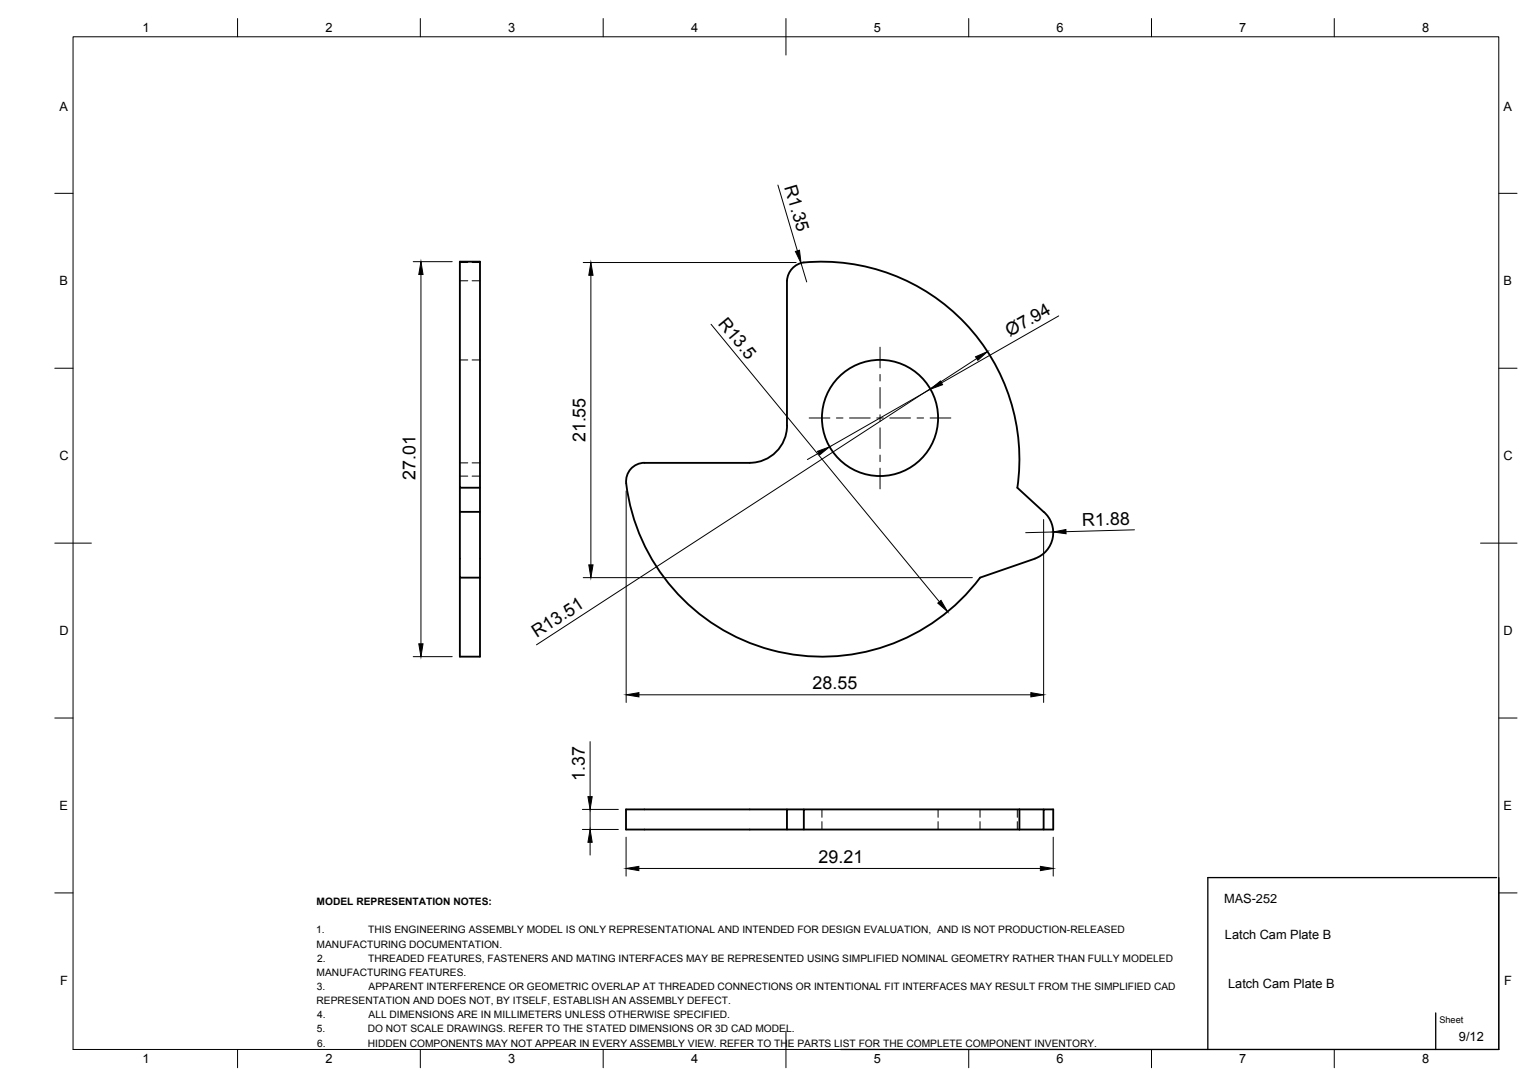
ISO-10303-21;
HEADER;
FILE_DESCRIPTION((''),'2;1');
FILE_NAME('Latch Cam Plate B.step','2026-10-06T07:01:46+05:00',(''),(''),'','','');
FILE_SCHEMA (('AUTOMOTIVE_DESIGN { 1 0 10303 214 3 1 1 }'));
ENDSEC;
DATA;
#10=MECHANICAL_DESIGN_GEOMETRIC_PRESENTATION_REPRESENTATION('',(#151),#11396);
#121=SHAPE_REPRESENTATION_RELATIONSHIP('SRR','None',#11468,#136) ;
#136=ADVANCED_BREP_SHAPE_REPRESENTATION('',(#166),#11394) ;
#151=STYLED_ITEM('',(#11552),#166) ;
#166=MANIFOLD_SOLID_BREP('Latch Cam Plate B',#5582) ;
#374=FACE_BOUND('',#1212,.T.) ;
#375=FACE_BOUND('',#1214,.T.) ;
#500=PLANE('',#6364) ;
#501=PLANE('',#6371) ;
#502=PLANE('',#6375) ;
#503=PLANE('',#6382) ;
#504=PLANE('',#6383) ;
#505=PLANE('',#6384) ;
#827=FACE_OUTER_BOUND('',#1200,.T.) ;
#828=FACE_OUTER_BOUND('',#1201,.T.) ;
#829=FACE_OUTER_BOUND('',#1202,.T.) ;
#830=FACE_OUTER_BOUND('',#1203,.T.) ;
#831=FACE_OUTER_BOUND('',#1204,.T.) ;
#832=FACE_OUTER_BOUND('',#1205,.T.) ;
#833=FACE_OUTER_BOUND('',#1206,.T.) ;
#834=FACE_OUTER_BOUND('',#1207,.T.) ;
#835=FACE_OUTER_BOUND('',#1208,.T.) ;
#836=FACE_OUTER_BOUND('',#1209,.T.) ;
#837=FACE_OUTER_BOUND('',#1210,.T.) ;
#838=FACE_OUTER_BOUND('',#1211,.T.) ;
#839=FACE_OUTER_BOUND('',#1213,.T.) ;
#1200=EDGE_LOOP('',(#5014,#5015,#5016,#5017)) ;
#1201=EDGE_LOOP('',(#5018,#5019,#5020,#5021)) ;
#1202=EDGE_LOOP('',(#5022,#5023,#5024,#5025)) ;
#1203=EDGE_LOOP('',(#5026,#5027,#5028,#5029)) ;
#1204=EDGE_LOOP('',(#5030,#5031,#5032,#5033)) ;
#1205=EDGE_LOOP('',(#5034,#5035,#5036,#5037)) ;
#1206=EDGE_LOOP('',(#5038,#5039,#5040,#5041)) ;
#1207=EDGE_LOOP('',(#5042,#5043,#5044,#5045)) ;
#1208=EDGE_LOOP('',(#5046,#5047,#5048,#5049)) ;
#1209=EDGE_LOOP('',(#5050,#5051,#5052,#5053)) ;
#1210=EDGE_LOOP('',(#5054,#5055,#5056,#5057)) ;
#1211=EDGE_LOOP('',(#5058,#5059,#5060,#5061,#5062,#5063,#5064,#5065,#5066,
#5067)) ;
#1212=EDGE_LOOP('',(#5068)) ;
#1213=EDGE_LOOP('',(#5069,#5070,#5071,#5072,#5073,#5074,#5075,#5076,#5077,
#5078)) ;
#1214=EDGE_LOOP('',(#5079)) ;
#1583=LINE('',#11263,#1966) ;
#1584=LINE('',#11270,#1967) ;
#1585=LINE('',#11273,#1968) ;
#1586=LINE('',#11276,#1969) ;
#1587=LINE('',#11278,#1970) ;
#1588=LINE('',#11279,#1971) ;
#1589=LINE('',#11285,#1972) ;
#1590=LINE('',#11291,#1973) ;
#1591=LINE('',#11294,#1974) ;
#1592=LINE('',#11296,#1975) ;
#1593=LINE('',#11297,#1976) ;
#1594=LINE('',#11303,#1977) ;
#1595=LINE('',#11306,#1978) ;
#1596=LINE('',#11308,#1979) ;
#1597=LINE('',#11309,#1980) ;
#1598=LINE('',#11315,#1981) ;
#1599=LINE('',#11321,#1982) ;
#1600=LINE('',#11323,#1983) ;
#1601=LINE('',#11324,#1984) ;
#1966=VECTOR('',#7997,3.97) ;
#1967=VECTOR('',#8004,10.) ;
#1968=VECTOR('',#8007,10.) ;
#1969=VECTOR('',#8010,10.) ;
#1970=VECTOR('',#8011,10.) ;
#1971=VECTOR('',#8012,10.) ;
#1972=VECTOR('',#8019,10.) ;
#1973=VECTOR('',#8026,10.) ;
#1974=VECTOR('',#8029,10.) ;
#1975=VECTOR('',#8030,10.) ;
#1976=VECTOR('',#8031,10.) ;
#1977=VECTOR('',#8038,10.) ;
#1978=VECTOR('',#8041,10.) ;
#1979=VECTOR('',#8042,10.) ;
#1980=VECTOR('',#8043,10.) ;
#1981=VECTOR('',#8050,10.) ;
#1982=VECTOR('',#8057,10.) ;
#1983=VECTOR('',#8060,10.) ;
#1984=VECTOR('',#8061,10.) ;
#2251=CIRCLE('',#6359,3.97) ;
#2252=CIRCLE('',#6360,3.97) ;
#2253=CIRCLE('',#6362,2.55000000000001) ;
#2254=CIRCLE('',#6363,2.55000000000001) ;
#2255=CIRCLE('',#6366,1.34638068543699) ;
#2256=CIRCLE('',#6367,1.34638068543699) ;
#2257=CIRCLE('',#6369,13.5130476224576) ;
#2258=CIRCLE('',#6370,13.5130476224576) ;
#2259=CIRCLE('',#6373,1.8820937834387) ;
#2260=CIRCLE('',#6374,1.8820937834387) ;
#2261=CIRCLE('',#6377,13.5002427920346) ;
#2262=CIRCLE('',#6378,13.5002427920346) ;
#2263=CIRCLE('',#6380,1.26348906976575) ;
#2264=CIRCLE('',#6381,1.26348906976575) ;
#2720=VERTEX_POINT('',#11260) ;
#2721=VERTEX_POINT('',#11262) ;
#2722=VERTEX_POINT('',#11266) ;
#2723=VERTEX_POINT('',#11267) ;
#2724=VERTEX_POINT('',#11269) ;
#2725=VERTEX_POINT('',#11271) ;
#2726=VERTEX_POINT('',#11275) ;
#2727=VERTEX_POINT('',#11277) ;
#2728=VERTEX_POINT('',#11281) ;
#2729=VERTEX_POINT('',#11283) ;
#2730=VERTEX_POINT('',#11287) ;
#2731=VERTEX_POINT('',#11289) ;
#2732=VERTEX_POINT('',#11293) ;
#2733=VERTEX_POINT('',#11295) ;
#2734=VERTEX_POINT('',#11299) ;
#2735=VERTEX_POINT('',#11301) ;
#2736=VERTEX_POINT('',#11305) ;
#2737=VERTEX_POINT('',#11307) ;
#2738=VERTEX_POINT('',#11311) ;
#2739=VERTEX_POINT('',#11313) ;
#2740=VERTEX_POINT('',#11317) ;
#2741=VERTEX_POINT('',#11319) ;
#3489=EDGE_CURVE('',#2720,#2720,#2251,.T.) ;
#3490=EDGE_CURVE('',#2720,#2721,#1583,.T.) ;
#3491=EDGE_CURVE('',#2721,#2721,#2252,.T.) ;
#3492=EDGE_CURVE('',#2722,#2723,#2253,.T.) ;
#3493=EDGE_CURVE('',#2722,#2724,#1584,.T.) ;
#3494=EDGE_CURVE('',#2725,#2724,#2254,.T.) ;
#3495=EDGE_CURVE('',#2723,#2725,#1585,.T.) ;
#3496=EDGE_CURVE('',#2726,#2723,#1586,.T.) ;
#3497=EDGE_CURVE('',#2727,#2725,#1587,.T.) ;
#3498=EDGE_CURVE('',#2726,#2727,#1588,.T.) ;
#3499=EDGE_CURVE('',#2728,#2726,#2255,.T.) ;
#3500=EDGE_CURVE('',#2729,#2727,#2256,.T.) ;
#3501=EDGE_CURVE('',#2728,#2729,#1589,.T.) ;
#3502=EDGE_CURVE('',#2730,#2728,#2257,.T.) ;
#3503=EDGE_CURVE('',#2731,#2729,#2258,.T.) ;
#3504=EDGE_CURVE('',#2730,#2731,#1590,.T.) ;
#3505=EDGE_CURVE('',#2732,#2730,#1591,.T.) ;
#3506=EDGE_CURVE('',#2733,#2731,#1592,.T.) ;
#3507=EDGE_CURVE('',#2732,#2733,#1593,.T.) ;
#3508=EDGE_CURVE('',#2734,#2732,#2259,.T.) ;
#3509=EDGE_CURVE('',#2735,#2733,#2260,.T.) ;
#3510=EDGE_CURVE('',#2734,#2735,#1594,.T.) ;
#3511=EDGE_CURVE('',#2736,#2734,#1595,.T.) ;
#3512=EDGE_CURVE('',#2737,#2735,#1596,.T.) ;
#3513=EDGE_CURVE('',#2736,#2737,#1597,.T.) ;
#3514=EDGE_CURVE('',#2738,#2736,#2261,.T.) ;
#3515=EDGE_CURVE('',#2739,#2737,#2262,.T.) ;
#3516=EDGE_CURVE('',#2738,#2739,#1598,.T.) ;
#3517=EDGE_CURVE('',#2740,#2738,#2263,.T.) ;
#3518=EDGE_CURVE('',#2741,#2739,#2264,.T.) ;
#3519=EDGE_CURVE('',#2740,#2741,#1599,.T.) ;
#3520=EDGE_CURVE('',#2722,#2740,#1600,.T.) ;
#3521=EDGE_CURVE('',#2724,#2741,#1601,.T.) ;
#5014=ORIENTED_EDGE('',*,*,#3489,.F.) ;
#5015=ORIENTED_EDGE('',*,*,#3490,.T.) ;
#5016=ORIENTED_EDGE('',*,*,#3491,.T.) ;
#5017=ORIENTED_EDGE('',*,*,#3490,.F.) ;
#5018=ORIENTED_EDGE('',*,*,#3492,.F.) ;
#5019=ORIENTED_EDGE('',*,*,#3493,.T.) ;
#5020=ORIENTED_EDGE('',*,*,#3494,.F.) ;
#5021=ORIENTED_EDGE('',*,*,#3495,.F.) ;
#5022=ORIENTED_EDGE('',*,*,#3496,.T.) ;
#5023=ORIENTED_EDGE('',*,*,#3495,.T.) ;
#5024=ORIENTED_EDGE('',*,*,#3497,.F.) ;
#5025=ORIENTED_EDGE('',*,*,#3498,.F.) ;
#5026=ORIENTED_EDGE('',*,*,#3499,.T.) ;
#5027=ORIENTED_EDGE('',*,*,#3498,.T.) ;
#5028=ORIENTED_EDGE('',*,*,#3500,.F.) ;
#5029=ORIENTED_EDGE('',*,*,#3501,.F.) ;
#5030=ORIENTED_EDGE('',*,*,#3502,.T.) ;
#5031=ORIENTED_EDGE('',*,*,#3501,.T.) ;
#5032=ORIENTED_EDGE('',*,*,#3503,.F.) ;
#5033=ORIENTED_EDGE('',*,*,#3504,.F.) ;
#5034=ORIENTED_EDGE('',*,*,#3505,.T.) ;
#5035=ORIENTED_EDGE('',*,*,#3504,.T.) ;
#5036=ORIENTED_EDGE('',*,*,#3506,.F.) ;
#5037=ORIENTED_EDGE('',*,*,#3507,.F.) ;
#5038=ORIENTED_EDGE('',*,*,#3508,.T.) ;
#5039=ORIENTED_EDGE('',*,*,#3507,.T.) ;
#5040=ORIENTED_EDGE('',*,*,#3509,.F.) ;
#5041=ORIENTED_EDGE('',*,*,#3510,.F.) ;
#5042=ORIENTED_EDGE('',*,*,#3511,.T.) ;
#5043=ORIENTED_EDGE('',*,*,#3510,.T.) ;
#5044=ORIENTED_EDGE('',*,*,#3512,.F.) ;
#5045=ORIENTED_EDGE('',*,*,#3513,.F.) ;
#5046=ORIENTED_EDGE('',*,*,#3514,.T.) ;
#5047=ORIENTED_EDGE('',*,*,#3513,.T.) ;
#5048=ORIENTED_EDGE('',*,*,#3515,.F.) ;
#5049=ORIENTED_EDGE('',*,*,#3516,.F.) ;
#5050=ORIENTED_EDGE('',*,*,#3517,.T.) ;
#5051=ORIENTED_EDGE('',*,*,#3516,.T.) ;
#5052=ORIENTED_EDGE('',*,*,#3518,.F.) ;
#5053=ORIENTED_EDGE('',*,*,#3519,.F.) ;
#5054=ORIENTED_EDGE('',*,*,#3520,.T.) ;
#5055=ORIENTED_EDGE('',*,*,#3519,.T.) ;
#5056=ORIENTED_EDGE('',*,*,#3521,.F.) ;
#5057=ORIENTED_EDGE('',*,*,#3493,.F.) ;
#5058=ORIENTED_EDGE('',*,*,#3521,.T.) ;
#5059=ORIENTED_EDGE('',*,*,#3518,.T.) ;
#5060=ORIENTED_EDGE('',*,*,#3515,.T.) ;
#5061=ORIENTED_EDGE('',*,*,#3512,.T.) ;
#5062=ORIENTED_EDGE('',*,*,#3509,.T.) ;
#5063=ORIENTED_EDGE('',*,*,#3506,.T.) ;
#5064=ORIENTED_EDGE('',*,*,#3503,.T.) ;
#5065=ORIENTED_EDGE('',*,*,#3500,.T.) ;
#5066=ORIENTED_EDGE('',*,*,#3497,.T.) ;
#5067=ORIENTED_EDGE('',*,*,#3494,.T.) ;
#5068=ORIENTED_EDGE('',*,*,#3489,.T.) ;
#5069=ORIENTED_EDGE('',*,*,#3520,.F.) ;
#5070=ORIENTED_EDGE('',*,*,#3492,.T.) ;
#5071=ORIENTED_EDGE('',*,*,#3496,.F.) ;
#5072=ORIENTED_EDGE('',*,*,#3499,.F.) ;
#5073=ORIENTED_EDGE('',*,*,#3502,.F.) ;
#5074=ORIENTED_EDGE('',*,*,#3505,.F.) ;
#5075=ORIENTED_EDGE('',*,*,#3508,.F.) ;
#5076=ORIENTED_EDGE('',*,*,#3511,.F.) ;
#5077=ORIENTED_EDGE('',*,*,#3514,.F.) ;
#5078=ORIENTED_EDGE('',*,*,#3517,.F.) ;
#5079=ORIENTED_EDGE('',*,*,#3491,.F.) ;
#5224=CYLINDRICAL_SURFACE('',#6358,3.97) ;
#5225=CYLINDRICAL_SURFACE('',#6361,2.55000000000001) ;
#5226=CYLINDRICAL_SURFACE('',#6365,1.34638068543699) ;
#5227=CYLINDRICAL_SURFACE('',#6368,13.5130476224576) ;
#5228=CYLINDRICAL_SURFACE('',#6372,1.8820937834387) ;
#5229=CYLINDRICAL_SURFACE('',#6376,13.5002427920346) ;
#5230=CYLINDRICAL_SURFACE('',#6379,1.26348906976575) ;
#5552=ADVANCED_FACE('',(#827),#5224,.F.) ;
#5553=ADVANCED_FACE('',(#828),#5225,.F.) ;
#5554=ADVANCED_FACE('',(#829),#500,.T.) ;
#5555=ADVANCED_FACE('',(#830),#5226,.T.) ;
#5556=ADVANCED_FACE('',(#831),#5227,.T.) ;
#5557=ADVANCED_FACE('',(#832),#501,.T.) ;
#5558=ADVANCED_FACE('',(#833),#5228,.T.) ;
#5559=ADVANCED_FACE('',(#834),#502,.T.) ;
#5560=ADVANCED_FACE('',(#835),#5229,.T.) ;
#5561=ADVANCED_FACE('',(#836),#5230,.T.) ;
#5562=ADVANCED_FACE('',(#837),#503,.T.) ;
#5563=ADVANCED_FACE('',(#838,#374),#504,.T.) ;
#5564=ADVANCED_FACE('',(#839,#375),#505,.F.) ;
#5582=CLOSED_SHELL('',(#5552,#5553,#5554,#5555,#5556,#5557,#5558,#5559,
#5560,#5561,#5562,#5563,#5564)) ;
#6357=AXIS2_PLACEMENT_3D('',#11258,#7991,#7992) ;
#6358=AXIS2_PLACEMENT_3D('',#11259,#7993,#7994) ;
#6359=AXIS2_PLACEMENT_3D('',#11261,#7995,#7996) ;
#6360=AXIS2_PLACEMENT_3D('',#11264,#7998,#7999) ;
#6361=AXIS2_PLACEMENT_3D('',#11265,#8000,#8001) ;
#6362=AXIS2_PLACEMENT_3D('',#11268,#8002,#8003) ;
#6363=AXIS2_PLACEMENT_3D('',#11272,#8005,#8006) ;
#6364=AXIS2_PLACEMENT_3D('',#11274,#8008,#8009) ;
#6365=AXIS2_PLACEMENT_3D('',#11280,#8013,#8014) ;
#6366=AXIS2_PLACEMENT_3D('',#11282,#8015,#8016) ;
#6367=AXIS2_PLACEMENT_3D('',#11284,#8017,#8018) ;
#6368=AXIS2_PLACEMENT_3D('',#11286,#8020,#8021) ;
#6369=AXIS2_PLACEMENT_3D('',#11288,#8022,#8023) ;
#6370=AXIS2_PLACEMENT_3D('',#11290,#8024,#8025) ;
#6371=AXIS2_PLACEMENT_3D('',#11292,#8027,#8028) ;
#6372=AXIS2_PLACEMENT_3D('',#11298,#8032,#8033) ;
#6373=AXIS2_PLACEMENT_3D('',#11300,#8034,#8035) ;
#6374=AXIS2_PLACEMENT_3D('',#11302,#8036,#8037) ;
#6375=AXIS2_PLACEMENT_3D('',#11304,#8039,#8040) ;
#6376=AXIS2_PLACEMENT_3D('',#11310,#8044,#8045) ;
#6377=AXIS2_PLACEMENT_3D('',#11312,#8046,#8047) ;
#6378=AXIS2_PLACEMENT_3D('',#11314,#8048,#8049) ;
#6379=AXIS2_PLACEMENT_3D('',#11316,#8051,#8052) ;
#6380=AXIS2_PLACEMENT_3D('',#11318,#8053,#8054) ;
#6381=AXIS2_PLACEMENT_3D('',#11320,#8055,#8056) ;
#6382=AXIS2_PLACEMENT_3D('',#11322,#8058,#8059) ;
#6383=AXIS2_PLACEMENT_3D('',#11325,#8062,#8063) ;
#6384=AXIS2_PLACEMENT_3D('',#11326,#8064,#8065) ;
#7991=DIRECTION('axis',(0.,0.,1.)) ;
#7992=DIRECTION('refdir',(1.,0.,0.)) ;
#7993=DIRECTION('center_axis',(1.,0.,0.)) ;
#7994=DIRECTION('ref_axis',(0.,0.,-1.)) ;
#7995=DIRECTION('center_axis',(-1.,0.,0.)) ;
#7996=DIRECTION('ref_axis',(0.,0.,-1.)) ;
#7997=DIRECTION('',(-1.,0.,0.)) ;
#7998=DIRECTION('center_axis',(-1.,0.,0.)) ;
#7999=DIRECTION('ref_axis',(0.,0.,-1.)) ;
#8000=DIRECTION('center_axis',(1.,0.,0.)) ;
#8001=DIRECTION('ref_axis',(0.,-1.,-6.96610525254997E-15)) ;
#8002=DIRECTION('center_axis',(1.,0.,0.)) ;
#8003=DIRECTION('ref_axis',(0.,-1.,-6.96610525254997E-15)) ;
#8004=DIRECTION('',(1.,0.,0.)) ;
#8005=DIRECTION('center_axis',(-1.,0.,0.)) ;
#8006=DIRECTION('ref_axis',(0.,-1.,-6.96610525254997E-15)) ;
#8007=DIRECTION('',(1.,0.,0.)) ;
#8008=DIRECTION('center_axis',(0.,0.,1.)) ;
#8009=DIRECTION('ref_axis',(0.,-1.,0.)) ;
#8010=DIRECTION('',(0.,-1.,0.)) ;
#8011=DIRECTION('',(0.,-1.,0.)) ;
#8012=DIRECTION('',(1.,0.,0.)) ;
#8013=DIRECTION('center_axis',(1.,0.,0.)) ;
#8014=DIRECTION('ref_axis',(0.,0.98957973940004,0.143985899896303)) ;
#8015=DIRECTION('center_axis',(1.,0.,0.)) ;
#8016=DIRECTION('ref_axis',(0.,0.98957973940004,0.143985899896303)) ;
#8017=DIRECTION('center_axis',(1.,0.,0.)) ;
#8018=DIRECTION('ref_axis',(0.,0.98957973940004,0.143985899896303)) ;
#8019=DIRECTION('',(1.,0.,0.)) ;
#8020=DIRECTION('center_axis',(1.,0.,0.)) ;
#8021=DIRECTION('ref_axis',(0.,-0.143772557860476,-0.98961075762456)) ;
#8022=DIRECTION('center_axis',(1.,0.,0.)) ;
#8023=DIRECTION('ref_axis',(0.,-0.143772557860476,-0.98961075762456)) ;
#8024=DIRECTION('center_axis',(1.,0.,0.)) ;
#8025=DIRECTION('ref_axis',(0.,-0.143772557860476,-0.98961075762456)) ;
#8026=DIRECTION('',(1.,0.,0.)) ;
#8027=DIRECTION('center_axis',(0.,0.737154140200741,-0.675724628517347)) ;
#8028=DIRECTION('ref_axis',(0.,0.675724628517347,0.737154140200741)) ;
#8029=DIRECTION('',(0.,0.675724628517346,0.737154140200741)) ;
#8030=DIRECTION('',(0.,0.675724628517346,0.737154140200741)) ;
#8031=DIRECTION('',(1.,0.,0.)) ;
#8032=DIRECTION('center_axis',(1.,0.,0.)) ;
#8033=DIRECTION('ref_axis',(0.,-0.942609625269263,-0.333896831895331)) ;
#8034=DIRECTION('center_axis',(1.,0.,0.)) ;
#8035=DIRECTION('ref_axis',(0.,-0.942609625269263,-0.333896831895331)) ;
#8036=DIRECTION('center_axis',(1.,0.,0.)) ;
#8037=DIRECTION('ref_axis',(0.,-0.942609625269263,-0.333896831895331)) ;
#8038=DIRECTION('',(1.,0.,0.)) ;
#8039=DIRECTION('center_axis',(0.,-0.944836198498626,-0.327543215479523)) ;
#8040=DIRECTION('ref_axis',(0.,0.327543215479523,-0.944836198498626)) ;
#8041=DIRECTION('',(0.,0.327543215479523,-0.944836198498626)) ;
#8042=DIRECTION('',(0.,0.327543215479523,-0.944836198498626)) ;
#8043=DIRECTION('',(1.,0.,0.)) ;
#8044=DIRECTION('center_axis',(1.,0.,0.)) ;
#8045=DIRECTION('ref_axis',(0.,-0.122163634017166,0.992509973009702)) ;
#8046=DIRECTION('center_axis',(1.,0.,0.)) ;
#8047=DIRECTION('ref_axis',(0.,-0.122163634017166,0.992509973009702)) ;
#8048=DIRECTION('center_axis',(1.,0.,0.)) ;
#8049=DIRECTION('ref_axis',(0.,-0.122163634017166,0.992509973009702)) ;
#8050=DIRECTION('',(1.,0.,0.)) ;
#8051=DIRECTION('center_axis',(1.,0.,0.)) ;
#8052=DIRECTION('ref_axis',(0.,0.999988378789617,0.00482102537998268)) ;
#8053=DIRECTION('center_axis',(1.,0.,0.)) ;
#8054=DIRECTION('ref_axis',(0.,0.999988378789617,0.00482102537998268)) ;
#8055=DIRECTION('center_axis',(1.,0.,0.)) ;
#8056=DIRECTION('ref_axis',(0.,0.999988378789617,0.00482102537998268)) ;
#8057=DIRECTION('',(1.,0.,0.)) ;
#8058=DIRECTION('center_axis',(0.,1.,0.)) ;
#8059=DIRECTION('ref_axis',(0.,0.,1.)) ;
#8060=DIRECTION('',(0.,0.,1.)) ;
#8061=DIRECTION('',(0.,0.,1.)) ;
#8062=DIRECTION('center_axis',(1.,0.,0.)) ;
#8063=DIRECTION('ref_axis',(0.,0.,-1.)) ;
#8064=DIRECTION('center_axis',(1.,0.,0.)) ;
#8065=DIRECTION('ref_axis',(0.,0.,-1.)) ;
#11258=CARTESIAN_POINT('',(0.,0.,0.)) ;
#11259=CARTESIAN_POINT('Origin',(4.1,17.565,27.14)) ;
#11260=CARTESIAN_POINT('',(5.47,17.565,31.11)) ;
#11261=CARTESIAN_POINT('Origin',(5.47,17.565,27.14)) ;
#11262=CARTESIAN_POINT('',(4.1,17.565,31.11)) ;
#11263=CARTESIAN_POINT('',(4.1,17.565,31.11)) ;
#11264=CARTESIAN_POINT('Origin',(4.1,17.565,27.14)) ;
#11265=CARTESIAN_POINT('Origin',(4.1,17.05,36.05)) ;
#11266=CARTESIAN_POINT('',(4.1,14.5,36.05)) ;
#11267=CARTESIAN_POINT('',(4.1,17.05,33.5)) ;
#11268=CARTESIAN_POINT('Origin',(4.1,17.05,36.05)) ;
#11269=CARTESIAN_POINT('',(5.47,14.5,36.05)) ;
#11270=CARTESIAN_POINT('',(4.1,14.5,36.05)) ;
#11271=CARTESIAN_POINT('',(5.47,17.05,33.5)) ;
#11272=CARTESIAN_POINT('Origin',(5.47,17.05,36.05)) ;
#11273=CARTESIAN_POINT('',(4.1,17.05,33.5)) ;
#11274=CARTESIAN_POINT('Origin',(4.1,26.95,33.5)) ;
#11275=CARTESIAN_POINT('',(4.1,26.95,33.5)) ;
#11276=CARTESIAN_POINT('',(4.1,26.95,33.5)) ;
#11277=CARTESIAN_POINT('',(5.47,26.95,33.5)) ;
#11278=CARTESIAN_POINT('',(5.47,26.95,33.5)) ;
#11279=CARTESIAN_POINT('',(4.1,26.95,33.5)) ;
#11280=CARTESIAN_POINT('Origin',(4.1,26.867648952172,32.1561401654044)) ;
#11281=CARTESIAN_POINT('',(4.1,28.2,32.35)) ;
#11282=CARTESIAN_POINT('Origin',(4.1,26.867648952172,32.1561401654044)) ;
#11283=CARTESIAN_POINT('',(5.47,28.2,32.35)) ;
#11284=CARTESIAN_POINT('Origin',(5.47,26.867648952172,32.1561401654044)) ;
#11285=CARTESIAN_POINT('',(4.1,28.2,32.35)) ;
#11286=CARTESIAN_POINT('Origin',(4.1,14.7428054211711,31.122657295477)) ;
#11287=CARTESIAN_POINT('',(4.1,12.8,17.75)) ;
#11288=CARTESIAN_POINT('Origin',(4.1,14.7428054211711,31.122657295477)) ;
#11289=CARTESIAN_POINT('',(5.47,12.8,17.75)) ;
#11290=CARTESIAN_POINT('Origin',(5.47,14.7428054211711,31.122657295477)) ;
#11291=CARTESIAN_POINT('',(4.1,12.8,17.75)) ;
#11292=CARTESIAN_POINT('Origin',(4.1,11.15,15.95)) ;
#11293=CARTESIAN_POINT('',(4.1,11.15,15.95)) ;
#11294=CARTESIAN_POINT('',(4.1,11.15,15.95)) ;
#11295=CARTESIAN_POINT('',(5.47,11.15,15.95)) ;
#11296=CARTESIAN_POINT('',(5.47,11.15,15.95)) ;
#11297=CARTESIAN_POINT('',(4.1,11.15,15.95)) ;
#11298=CARTESIAN_POINT('Origin',(4.1,9.72407971592876,17.1784251516201)) ;
#11299=CARTESIAN_POINT('',(4.1,7.95,16.55)) ;
#11300=CARTESIAN_POINT('Origin',(4.1,9.72407971592876,17.1784251516201)) ;
#11301=CARTESIAN_POINT('',(5.47,7.95,16.55)) ;
#11302=CARTESIAN_POINT('Origin',(5.47,9.72407971592876,17.1784251516201)) ;
#11303=CARTESIAN_POINT('',(4.1,7.95,16.55)) ;
#11304=CARTESIAN_POINT('Origin',(4.1,6.65,20.3)) ;
#11305=CARTESIAN_POINT('',(4.1,6.65,20.3)) ;
#11306=CARTESIAN_POINT('',(4.1,6.65,20.3)) ;
#11307=CARTESIAN_POINT('',(5.47,6.65,20.3)) ;
#11308=CARTESIAN_POINT('',(5.47,6.65,20.3)) ;
#11309=CARTESIAN_POINT('',(4.1,6.65,20.3)) ;
#11310=CARTESIAN_POINT('Origin',(4.1,14.749238719589,31.1008743908533)) ;
#11311=CARTESIAN_POINT('',(4.1,13.1,44.5)) ;
#11312=CARTESIAN_POINT('Origin',(4.1,14.749238719589,31.1008743908533)) ;
#11313=CARTESIAN_POINT('',(5.47,13.1,44.5)) ;
#11314=CARTESIAN_POINT('Origin',(5.47,14.749238719589,31.1008743908533)) ;
#11315=CARTESIAN_POINT('',(4.1,13.1,44.5)) ;
#11316=CARTESIAN_POINT('Origin',(4.1,13.2365256135065,43.2439086871273)) ;
#11317=CARTESIAN_POINT('',(4.1,14.5,43.25)) ;
#11318=CARTESIAN_POINT('Origin',(4.1,13.2365256135065,43.2439086871273)) ;
#11319=CARTESIAN_POINT('',(5.47,14.5,43.25)) ;
#11320=CARTESIAN_POINT('Origin',(5.47,13.2365256135065,43.2439086871273)) ;
#11321=CARTESIAN_POINT('',(4.1,14.5,43.25)) ;
#11322=CARTESIAN_POINT('Origin',(4.1,14.5,36.05)) ;
#11323=CARTESIAN_POINT('',(4.1,14.5,36.05)) ;
#11324=CARTESIAN_POINT('',(5.47,14.5,36.05)) ;
#11325=CARTESIAN_POINT('Origin',(5.47,14.7524244855916,29.9018645625372)) ;
#11326=CARTESIAN_POINT('Origin',(4.1,14.7524244855916,29.9018645625372)) ;
#11377=UNCERTAINTY_MEASURE_WITH_UNIT(LENGTH_MEASURE(0.01),#11397,
'DISTANCE_ACCURACY_VALUE',
'Maximum model space distance between geometric entities at asserted c
onnectivities') ;
#11379=UNCERTAINTY_MEASURE_WITH_UNIT(LENGTH_MEASURE(0.01),#11397,
'DISTANCE_ACCURACY_VALUE',
'Maximum model space distance between geometric entities at asserted c
onnectivities') ;
#11394=(
GEOMETRIC_REPRESENTATION_CONTEXT(3)
GLOBAL_UNCERTAINTY_ASSIGNED_CONTEXT((#11377))
GLOBAL_UNIT_ASSIGNED_CONTEXT((#11397,#11399,#11400))
REPRESENTATION_CONTEXT('','3D')
) ;
#11396=(
GEOMETRIC_REPRESENTATION_CONTEXT(3)
GLOBAL_UNCERTAINTY_ASSIGNED_CONTEXT((#11379))
GLOBAL_UNIT_ASSIGNED_CONTEXT((#11397,#11399,#11400))
REPRESENTATION_CONTEXT('','3D')
) ;
#11397=(
LENGTH_UNIT()
NAMED_UNIT(*)
SI_UNIT(.MILLI.,.METRE.)
) ;
#11399=(
NAMED_UNIT(*)
PLANE_ANGLE_UNIT()
SI_UNIT($,.RADIAN.)
) ;
#11400=(
NAMED_UNIT(*)
SI_UNIT($,.STERADIAN.)
SOLID_ANGLE_UNIT()
) ;
#11415=SHAPE_DEFINITION_REPRESENTATION(#11431,#11468) ;
#11431=PRODUCT_DEFINITION_SHAPE('',$,#11485) ;
#11468=SHAPE_REPRESENTATION('',(#6357),#11394) ;
#11470=PRODUCT_DEFINITION_CONTEXT('part definition',#11520,'design') ;
#11485=PRODUCT_DEFINITION('Latch Cam Plate B','Latch Cam Plate B',
#11501,#11470) ;
#11501=PRODUCT_DEFINITION_FORMATION('',$,#11536) ;
#11520=APPLICATION_CONTEXT(
'Core Data for Automotive Mechanical Design Process') ;
#11521=PRODUCT_CONTEXT('part definition',#11520,'mechanical') ;
#11536=PRODUCT('Latch Cam Plate B','Latch Cam Plate B',$,(#11521)) ;
#11552=PRESENTATION_STYLE_ASSIGNMENT((#11568)) ;
#11568=SURFACE_STYLE_USAGE(.BOTH.,#11584) ;
#11584=SURFACE_SIDE_STYLE('',(#11600)) ;
#11600=SURFACE_STYLE_FILL_AREA(#11616) ;
#11616=FILL_AREA_STYLE('MAS-252 Metallic - Latch Cam Plate B',(#11632)) ;
#11632=FILL_AREA_STYLE_COLOUR('MAS-252 Metallic - Latch Cam Plate B',#11648) ;
#11648=COLOUR_RGB('MAS-252 Metallic - Latch Cam Plate B', 0.66274510, 0.83137255, 0.94901961) ;
ENDSEC;
END-ISO-10303-21;
